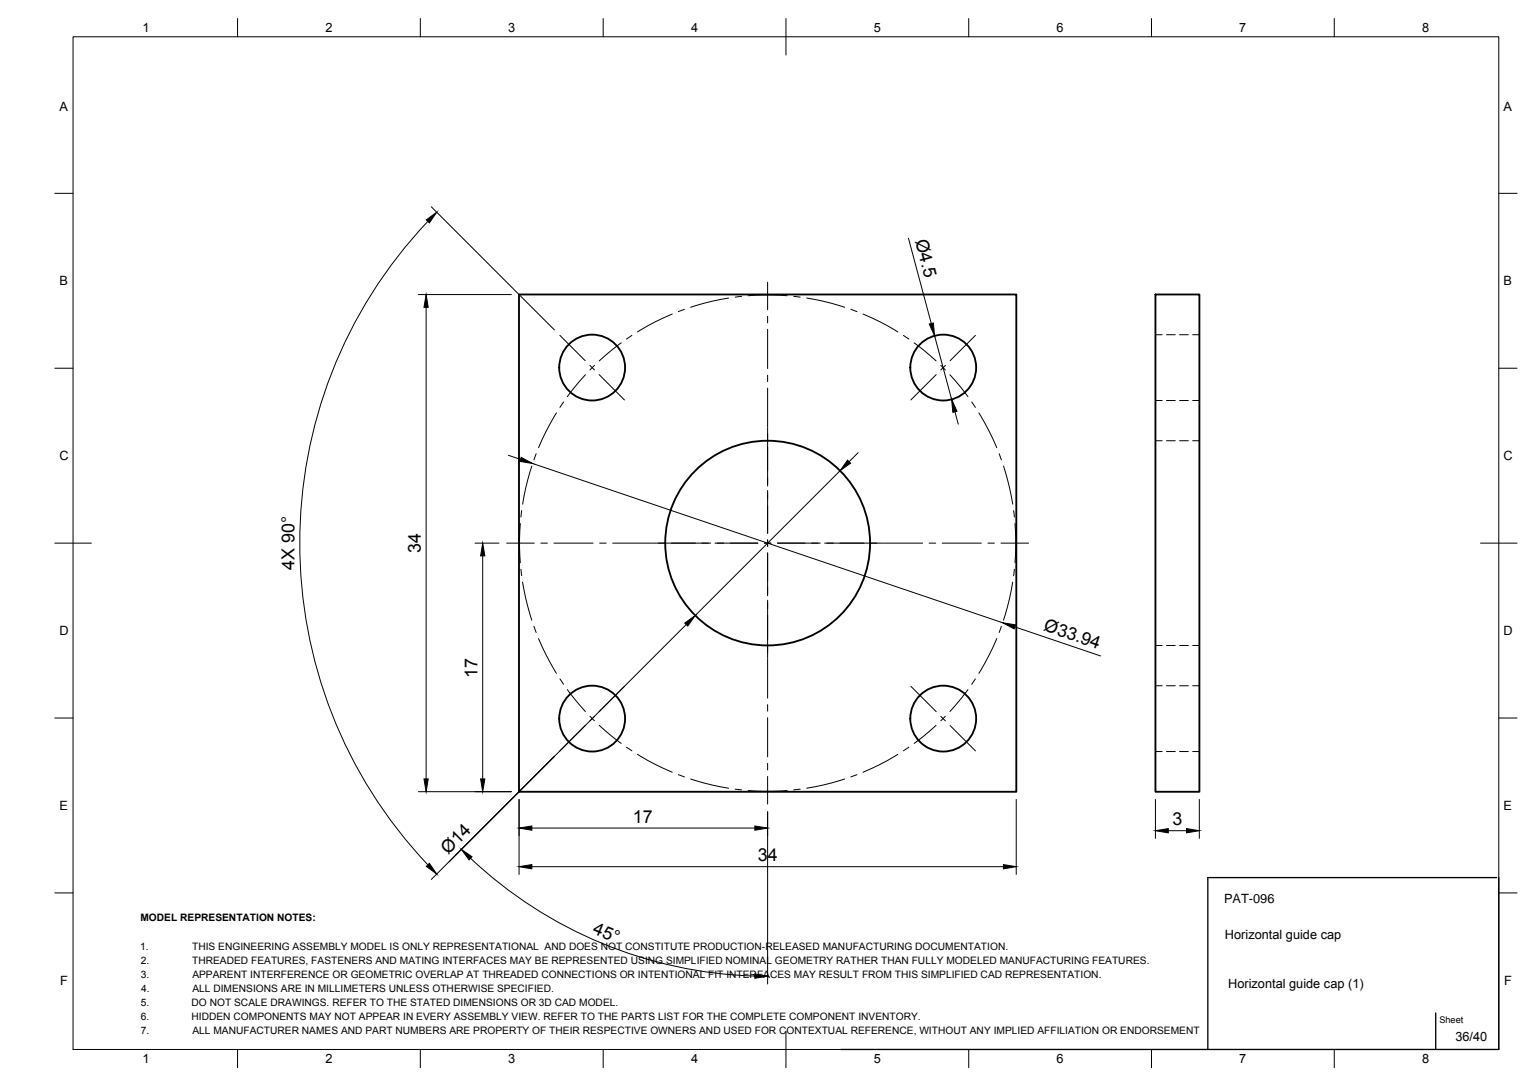
ISO-10303-21;
HEADER;
/* Generated by software containing ST-Developer
 * from STEP Tools, Inc. (www.steptools.com) 
 */

FILE_DESCRIPTION(
/* description */ ('PAT-096'),
/* implementation_level */ '2;1');

FILE_NAME(
/* name */ 'Horizontal guide cap.step',
/* time_stamp */ '2026-10-29T17:03:14-07:00',
/* author */ (''),
/* organization */ (''),
/* preprocessor_version */ 'ST-DEVELOPER v20.2',
/* originating_system */ 'Autodesk Translation Framework v15.17.0.0',
/* authorisation */ '');

FILE_SCHEMA (('AUTOMOTIVE_DESIGN { 1 0 10303 214 3 1 1 }'));
ENDSEC;

DATA;
#10=MECHANICAL_DESIGN_GEOMETRIC_PRESENTATION_REPRESENTATION('',(#433),#10650);
#363=SHAPE_REPRESENTATION_RELATIONSHIP('SRR','None',#10828,#394);
#394=ADVANCED_BREP_SHAPE_REPRESENTATION('',(#470),#10646);
#433=STYLED_ITEM('',(#11057),#470);
#470=MANIFOLD_SOLID_BREP('Body1',#5568);
#597=FACE_BOUND('',#1558,.T.);
#598=FACE_BOUND('',#1559,.T.);
#599=FACE_BOUND('',#1560,.T.);
#600=FACE_BOUND('',#1561,.T.);
#601=FACE_BOUND('',#1562,.T.);
#602=FACE_BOUND('',#1565,.T.);
#603=FACE_BOUND('',#1566,.T.);
#604=FACE_BOUND('',#1567,.T.);
#605=FACE_BOUND('',#1568,.T.);
#606=FACE_BOUND('',#1569,.T.);
#769=PLANE('',#6570);
#770=PLANE('',#6571);
#771=PLANE('',#6572);
#772=PLANE('',#6573);
#773=PLANE('',#6574);
#774=PLANE('',#6575);
#1091=FACE_OUTER_BOUND('',#1551,.T.);
#1092=FACE_OUTER_BOUND('',#1552,.T.);
#1093=FACE_OUTER_BOUND('',#1553,.T.);
#1094=FACE_OUTER_BOUND('',#1554,.T.);
#1095=FACE_OUTER_BOUND('',#1555,.T.);
#1096=FACE_OUTER_BOUND('',#1556,.T.);
#1097=FACE_OUTER_BOUND('',#1557,.T.);
#1098=FACE_OUTER_BOUND('',#1563,.T.);
#1099=FACE_OUTER_BOUND('',#1564,.T.);
#1100=FACE_OUTER_BOUND('',#1570,.T.);
#1101=FACE_OUTER_BOUND('',#1571,.T.);
#1551=EDGE_LOOP('',(#4935,#4936,#4937,#4938));
#1552=EDGE_LOOP('',(#4939,#4940,#4941,#4942));
#1553=EDGE_LOOP('',(#4943,#4944,#4945,#4946));
#1554=EDGE_LOOP('',(#4947,#4948,#4949,#4950));
#1555=EDGE_LOOP('',(#4951,#4952,#4953,#4954));
#1556=EDGE_LOOP('',(#4955,#4956,#4957,#4958));
#1557=EDGE_LOOP('',(#4959,#4960,#4961,#4962));
#1558=EDGE_LOOP('',(#4963));
#1559=EDGE_LOOP('',(#4964));
#1560=EDGE_LOOP('',(#4965));
#1561=EDGE_LOOP('',(#4966));
#1562=EDGE_LOOP('',(#4967));
#1563=EDGE_LOOP('',(#4968,#4969,#4970,#4971));
#1564=EDGE_LOOP('',(#4972,#4973,#4974,#4975));
#1565=EDGE_LOOP('',(#4976));
#1566=EDGE_LOOP('',(#4977));
#1567=EDGE_LOOP('',(#4978));
#1568=EDGE_LOOP('',(#4979));
#1569=EDGE_LOOP('',(#4980));
#1570=EDGE_LOOP('',(#4981,#4982,#4983,#4984));
#1571=EDGE_LOOP('',(#4985,#4986,#4987,#4988));
#1886=LINE('',#10372,#2215);
#1887=LINE('',#10378,#2216);
#1888=LINE('',#10384,#2217);
#1889=LINE('',#10390,#2218);
#1890=LINE('',#10396,#2219);
#1891=LINE('',#10401,#2220);
#1892=LINE('',#10403,#2221);
#1893=LINE('',#10405,#2222);
#1894=LINE('',#10406,#2223);
#1895=LINE('',#10409,#2224);
#1896=LINE('',#10411,#2225);
#1897=LINE('',#10412,#2226);
#1898=LINE('',#10415,#2227);
#1899=LINE('',#10417,#2228);
#1900=LINE('',#10418,#2229);
#1901=LINE('',#10420,#2230);
#1902=LINE('',#10421,#2231);
#2215=VECTOR('',#8240,0.225);
#2216=VECTOR('',#8247,0.225);
#2217=VECTOR('',#8254,0.225);
#2218=VECTOR('',#8261,0.225);
#2219=VECTOR('',#8268,0.7);
#2220=VECTOR('',#8273,1.);
#2221=VECTOR('',#8274,1.);
#2222=VECTOR('',#8275,1.);
#2223=VECTOR('',#8276,1.);
#2224=VECTOR('',#8279,1.);
#2225=VECTOR('',#8280,1.);
#2226=VECTOR('',#8281,1.);
#2227=VECTOR('',#8284,1.);
#2228=VECTOR('',#8285,1.);
#2229=VECTOR('',#8286,1.);
#2230=VECTOR('',#8289,1.);
#2231=VECTOR('',#8290,1.);
#2553=CIRCLE('',#6556,0.225);
#2554=CIRCLE('',#6557,0.225);
#2555=CIRCLE('',#6559,0.225);
#2556=CIRCLE('',#6560,0.225);
#2557=CIRCLE('',#6562,0.225);
#2558=CIRCLE('',#6563,0.225);
#2559=CIRCLE('',#6565,0.225);
#2560=CIRCLE('',#6566,0.225);
#2561=CIRCLE('',#6568,0.7);
#2562=CIRCLE('',#6569,0.7);
#2991=VERTEX_POINT('',#10369);
#2992=VERTEX_POINT('',#10371);
#2993=VERTEX_POINT('',#10375);
#2994=VERTEX_POINT('',#10377);
#2995=VERTEX_POINT('',#10381);
#2996=VERTEX_POINT('',#10383);
#2997=VERTEX_POINT('',#10387);
#2998=VERTEX_POINT('',#10389);
#2999=VERTEX_POINT('',#10393);
#3000=VERTEX_POINT('',#10395);
#3001=VERTEX_POINT('',#10399);
#3002=VERTEX_POINT('',#10400);
#3003=VERTEX_POINT('',#10402);
#3004=VERTEX_POINT('',#10404);
#3005=VERTEX_POINT('',#10408);
#3006=VERTEX_POINT('',#10410);
#3007=VERTEX_POINT('',#10414);
#3008=VERTEX_POINT('',#10416);
#3646=EDGE_CURVE('',#2991,#2991,#2553,.T.);
#3647=EDGE_CURVE('',#2991,#2992,#1886,.T.);
#3648=EDGE_CURVE('',#2992,#2992,#2554,.T.);
#3649=EDGE_CURVE('',#2993,#2993,#2555,.T.);
#3650=EDGE_CURVE('',#2993,#2994,#1887,.T.);
#3651=EDGE_CURVE('',#2994,#2994,#2556,.T.);
#3652=EDGE_CURVE('',#2995,#2995,#2557,.T.);
#3653=EDGE_CURVE('',#2995,#2996,#1888,.T.);
#3654=EDGE_CURVE('',#2996,#2996,#2558,.T.);
#3655=EDGE_CURVE('',#2997,#2997,#2559,.T.);
#3656=EDGE_CURVE('',#2997,#2998,#1889,.T.);
#3657=EDGE_CURVE('',#2998,#2998,#2560,.T.);
#3658=EDGE_CURVE('',#2999,#2999,#2561,.T.);
#3659=EDGE_CURVE('',#2999,#3000,#1890,.T.);
#3660=EDGE_CURVE('',#3000,#3000,#2562,.T.);
#3661=EDGE_CURVE('',#3001,#3002,#1891,.T.);
#3662=EDGE_CURVE('',#3002,#3003,#1892,.T.);
#3663=EDGE_CURVE('',#3004,#3003,#1893,.T.);
#3664=EDGE_CURVE('',#3001,#3004,#1894,.T.);
#3665=EDGE_CURVE('',#3005,#3001,#1895,.T.);
#3666=EDGE_CURVE('',#3006,#3004,#1896,.T.);
#3667=EDGE_CURVE('',#3005,#3006,#1897,.T.);
#3668=EDGE_CURVE('',#3007,#3005,#1898,.T.);
#3669=EDGE_CURVE('',#3008,#3006,#1899,.T.);
#3670=EDGE_CURVE('',#3007,#3008,#1900,.T.);
#3671=EDGE_CURVE('',#3002,#3007,#1901,.T.);
#3672=EDGE_CURVE('',#3003,#3008,#1902,.T.);
#4935=ORIENTED_EDGE('',*,*,#3646,.F.);
#4936=ORIENTED_EDGE('',*,*,#3647,.T.);
#4937=ORIENTED_EDGE('',*,*,#3648,.F.);
#4938=ORIENTED_EDGE('',*,*,#3647,.F.);
#4939=ORIENTED_EDGE('',*,*,#3649,.F.);
#4940=ORIENTED_EDGE('',*,*,#3650,.T.);
#4941=ORIENTED_EDGE('',*,*,#3651,.F.);
#4942=ORIENTED_EDGE('',*,*,#3650,.F.);
#4943=ORIENTED_EDGE('',*,*,#3652,.F.);
#4944=ORIENTED_EDGE('',*,*,#3653,.T.);
#4945=ORIENTED_EDGE('',*,*,#3654,.F.);
#4946=ORIENTED_EDGE('',*,*,#3653,.F.);
#4947=ORIENTED_EDGE('',*,*,#3655,.F.);
#4948=ORIENTED_EDGE('',*,*,#3656,.T.);
#4949=ORIENTED_EDGE('',*,*,#3657,.F.);
#4950=ORIENTED_EDGE('',*,*,#3656,.F.);
#4951=ORIENTED_EDGE('',*,*,#3658,.F.);
#4952=ORIENTED_EDGE('',*,*,#3659,.T.);
#4953=ORIENTED_EDGE('',*,*,#3660,.F.);
#4954=ORIENTED_EDGE('',*,*,#3659,.F.);
#4955=ORIENTED_EDGE('',*,*,#3661,.T.);
#4956=ORIENTED_EDGE('',*,*,#3662,.T.);
#4957=ORIENTED_EDGE('',*,*,#3663,.F.);
#4958=ORIENTED_EDGE('',*,*,#3664,.F.);
#4959=ORIENTED_EDGE('',*,*,#3665,.T.);
#4960=ORIENTED_EDGE('',*,*,#3664,.T.);
#4961=ORIENTED_EDGE('',*,*,#3666,.F.);
#4962=ORIENTED_EDGE('',*,*,#3667,.F.);
#4963=ORIENTED_EDGE('',*,*,#3660,.T.);
#4964=ORIENTED_EDGE('',*,*,#3657,.T.);
#4965=ORIENTED_EDGE('',*,*,#3654,.T.);
#4966=ORIENTED_EDGE('',*,*,#3651,.T.);
#4967=ORIENTED_EDGE('',*,*,#3648,.T.);
#4968=ORIENTED_EDGE('',*,*,#3668,.T.);
#4969=ORIENTED_EDGE('',*,*,#3667,.T.);
#4970=ORIENTED_EDGE('',*,*,#3669,.F.);
#4971=ORIENTED_EDGE('',*,*,#3670,.F.);
#4972=ORIENTED_EDGE('',*,*,#3671,.T.);
#4973=ORIENTED_EDGE('',*,*,#3670,.T.);
#4974=ORIENTED_EDGE('',*,*,#3672,.F.);
#4975=ORIENTED_EDGE('',*,*,#3662,.F.);
#4976=ORIENTED_EDGE('',*,*,#3658,.T.);
#4977=ORIENTED_EDGE('',*,*,#3655,.T.);
#4978=ORIENTED_EDGE('',*,*,#3652,.T.);
#4979=ORIENTED_EDGE('',*,*,#3649,.T.);
#4980=ORIENTED_EDGE('',*,*,#3646,.T.);
#4981=ORIENTED_EDGE('',*,*,#3672,.T.);
#4982=ORIENTED_EDGE('',*,*,#3669,.T.);
#4983=ORIENTED_EDGE('',*,*,#3666,.T.);
#4984=ORIENTED_EDGE('',*,*,#3663,.T.);
#4985=ORIENTED_EDGE('',*,*,#3671,.F.);
#4986=ORIENTED_EDGE('',*,*,#3661,.F.);
#4987=ORIENTED_EDGE('',*,*,#3665,.F.);
#4988=ORIENTED_EDGE('',*,*,#3668,.F.);
#5184=CYLINDRICAL_SURFACE('',#6555,0.225);
#5185=CYLINDRICAL_SURFACE('',#6558,0.225);
#5186=CYLINDRICAL_SURFACE('',#6561,0.225);
#5187=CYLINDRICAL_SURFACE('',#6564,0.225);
#5188=CYLINDRICAL_SURFACE('',#6567,0.7);
#5496=ADVANCED_FACE('',(#1091),#5184,.F.);
#5497=ADVANCED_FACE('',(#1092),#5185,.F.);
#5498=ADVANCED_FACE('',(#1093),#5186,.F.);
#5499=ADVANCED_FACE('',(#1094),#5187,.F.);
#5500=ADVANCED_FACE('',(#1095),#5188,.F.);
#5501=ADVANCED_FACE('',(#1096),#769,.T.);
#5502=ADVANCED_FACE('',(#1097,#597,#598,#599,#600,#601),#770,.T.);
#5503=ADVANCED_FACE('',(#1098),#771,.T.);
#5504=ADVANCED_FACE('',(#1099,#602,#603,#604,#605,#606),#772,.T.);
#5505=ADVANCED_FACE('',(#1100),#773,.T.);
#5506=ADVANCED_FACE('',(#1101),#774,.F.);
#5568=CLOSED_SHELL('',(#5496,#5497,#5498,#5499,#5500,#5501,#5502,#5503,
#5504,#5505,#5506));
#6554=AXIS2_PLACEMENT_3D('',#10367,#8234,#8235);
#6555=AXIS2_PLACEMENT_3D('',#10368,#8236,#8237);
#6556=AXIS2_PLACEMENT_3D('',#10370,#8238,#8239);
#6557=AXIS2_PLACEMENT_3D('',#10373,#8241,#8242);
#6558=AXIS2_PLACEMENT_3D('',#10374,#8243,#8244);
#6559=AXIS2_PLACEMENT_3D('',#10376,#8245,#8246);
#6560=AXIS2_PLACEMENT_3D('',#10379,#8248,#8249);
#6561=AXIS2_PLACEMENT_3D('',#10380,#8250,#8251);
#6562=AXIS2_PLACEMENT_3D('',#10382,#8252,#8253);
#6563=AXIS2_PLACEMENT_3D('',#10385,#8255,#8256);
#6564=AXIS2_PLACEMENT_3D('',#10386,#8257,#8258);
#6565=AXIS2_PLACEMENT_3D('',#10388,#8259,#8260);
#6566=AXIS2_PLACEMENT_3D('',#10391,#8262,#8263);
#6567=AXIS2_PLACEMENT_3D('',#10392,#8264,#8265);
#6568=AXIS2_PLACEMENT_3D('',#10394,#8266,#8267);
#6569=AXIS2_PLACEMENT_3D('',#10397,#8269,#8270);
#6570=AXIS2_PLACEMENT_3D('',#10398,#8271,#8272);
#6571=AXIS2_PLACEMENT_3D('',#10407,#8277,#8278);
#6572=AXIS2_PLACEMENT_3D('',#10413,#8282,#8283);
#6573=AXIS2_PLACEMENT_3D('',#10419,#8287,#8288);
#6574=AXIS2_PLACEMENT_3D('',#10422,#8291,#8292);
#6575=AXIS2_PLACEMENT_3D('',#10423,#8293,#8294);
#8234=DIRECTION('axis',(0.,0.,1.));
#8235=DIRECTION('refdir',(1.,0.,0.));
#8236=DIRECTION('center_axis',(1.,0.,0.));
#8237=DIRECTION('ref_axis',(0.,0.,-1.));
#8238=DIRECTION('center_axis',(1.,0.,0.));
#8239=DIRECTION('ref_axis',(0.,0.,-1.));
#8240=DIRECTION('',(1.,0.,0.));
#8241=DIRECTION('center_axis',(-1.,0.,0.));
#8242=DIRECTION('ref_axis',(0.,0.,-1.));
#8243=DIRECTION('center_axis',(1.,0.,0.));
#8244=DIRECTION('ref_axis',(0.,0.,-1.));
#8245=DIRECTION('center_axis',(1.,0.,0.));
#8246=DIRECTION('ref_axis',(0.,0.,-1.));
#8247=DIRECTION('',(1.,0.,0.));
#8248=DIRECTION('center_axis',(-1.,0.,0.));
#8249=DIRECTION('ref_axis',(0.,0.,-1.));
#8250=DIRECTION('center_axis',(1.,0.,0.));
#8251=DIRECTION('ref_axis',(0.,0.,-1.));
#8252=DIRECTION('center_axis',(1.,0.,0.));
#8253=DIRECTION('ref_axis',(0.,0.,-1.));
#8254=DIRECTION('',(1.,0.,0.));
#8255=DIRECTION('center_axis',(-1.,0.,0.));
#8256=DIRECTION('ref_axis',(0.,0.,-1.));
#8257=DIRECTION('center_axis',(1.,0.,0.));
#8258=DIRECTION('ref_axis',(0.,0.,-1.));
#8259=DIRECTION('center_axis',(1.,0.,0.));
#8260=DIRECTION('ref_axis',(0.,0.,-1.));
#8261=DIRECTION('',(1.,0.,0.));
#8262=DIRECTION('center_axis',(-1.,0.,0.));
#8263=DIRECTION('ref_axis',(0.,0.,-1.));
#8264=DIRECTION('center_axis',(1.,0.,0.));
#8265=DIRECTION('ref_axis',(0.,0.,-1.));
#8266=DIRECTION('center_axis',(1.,0.,0.));
#8267=DIRECTION('ref_axis',(0.,0.,-1.));
#8268=DIRECTION('',(1.,0.,0.));
#8269=DIRECTION('center_axis',(-1.,0.,0.));
#8270=DIRECTION('ref_axis',(0.,0.,-1.));
#8271=DIRECTION('center_axis',(0.,1.,0.));
#8272=DIRECTION('ref_axis',(-1.,0.,0.));
#8273=DIRECTION('',(-1.,0.,0.));
#8274=DIRECTION('',(0.,0.,1.));
#8275=DIRECTION('',(-1.,0.,0.));
#8276=DIRECTION('',(0.,0.,1.));
#8277=DIRECTION('center_axis',(1.,0.,0.));
#8278=DIRECTION('ref_axis',(0.,1.,0.));
#8279=DIRECTION('',(0.,1.,0.));
#8280=DIRECTION('',(0.,1.,0.));
#8281=DIRECTION('',(0.,0.,1.));
#8282=DIRECTION('center_axis',(0.,-1.,0.));
#8283=DIRECTION('ref_axis',(1.,0.,0.));
#8284=DIRECTION('',(1.,0.,0.));
#8285=DIRECTION('',(1.,0.,0.));
#8286=DIRECTION('',(0.,0.,1.));
#8287=DIRECTION('center_axis',(-1.,0.,0.));
#8288=DIRECTION('ref_axis',(0.,-1.,0.));
#8289=DIRECTION('',(0.,-1.,0.));
#8290=DIRECTION('',(0.,-1.,0.));
#8291=DIRECTION('center_axis',(0.,0.,1.));
#8292=DIRECTION('ref_axis',(1.,0.,0.));
#8293=DIRECTION('center_axis',(0.,0.,1.));
#8294=DIRECTION('ref_axis',(1.,0.,0.));
#10367=CARTESIAN_POINT('',(0.,0.,0.));
#10368=CARTESIAN_POINT('Origin',(8.1,3.2,2.8));
#10369=CARTESIAN_POINT('',(8.2,3.2,3.025));
#10370=CARTESIAN_POINT('Origin',(8.2,3.2,2.8));
#10371=CARTESIAN_POINT('',(8.5,3.2,3.025));
#10372=CARTESIAN_POINT('',(8.1,3.2,3.025));
#10373=CARTESIAN_POINT('Origin',(8.5,3.2,2.8));
#10374=CARTESIAN_POINT('Origin',(8.1,0.8,5.2));
#10375=CARTESIAN_POINT('',(8.2,0.8,5.425));
#10376=CARTESIAN_POINT('Origin',(8.2,0.8,5.2));
#10377=CARTESIAN_POINT('',(8.5,0.8,5.425));
#10378=CARTESIAN_POINT('',(8.1,0.8,5.425));
#10379=CARTESIAN_POINT('Origin',(8.5,0.8,5.2));
#10380=CARTESIAN_POINT('Origin',(8.1,0.8,2.8));
#10381=CARTESIAN_POINT('',(8.2,0.8,3.025));
#10382=CARTESIAN_POINT('Origin',(8.2,0.8,2.8));
#10383=CARTESIAN_POINT('',(8.5,0.8,3.025));
#10384=CARTESIAN_POINT('',(8.1,0.8,3.025));
#10385=CARTESIAN_POINT('Origin',(8.5,0.8,2.8));
#10386=CARTESIAN_POINT('Origin',(8.1,3.2,5.2));
#10387=CARTESIAN_POINT('',(8.2,3.2,5.425));
#10388=CARTESIAN_POINT('Origin',(8.2,3.2,5.2));
#10389=CARTESIAN_POINT('',(8.5,3.2,5.425));
#10390=CARTESIAN_POINT('',(8.1,3.2,5.425));
#10391=CARTESIAN_POINT('Origin',(8.5,3.2,5.2));
#10392=CARTESIAN_POINT('Origin',(8.1,2.,4.));
#10393=CARTESIAN_POINT('',(8.2,2.,4.7));
#10394=CARTESIAN_POINT('Origin',(8.2,2.,4.));
#10395=CARTESIAN_POINT('',(8.5,2.,4.7));
#10396=CARTESIAN_POINT('',(8.1,2.,4.7));
#10397=CARTESIAN_POINT('Origin',(8.5,2.,4.));
#10398=CARTESIAN_POINT('Origin',(8.5,3.7,2.3));
#10399=CARTESIAN_POINT('',(8.5,3.7,2.3));
#10400=CARTESIAN_POINT('',(8.2,3.7,2.3));
#10401=CARTESIAN_POINT('',(8.5,3.7,2.3));
#10402=CARTESIAN_POINT('',(8.2,3.7,5.7));
#10403=CARTESIAN_POINT('',(8.2,3.7,2.3));
#10404=CARTESIAN_POINT('',(8.5,3.7,5.7));
#10405=CARTESIAN_POINT('',(8.5,3.7,5.7));
#10406=CARTESIAN_POINT('',(8.5,3.7,2.3));
#10407=CARTESIAN_POINT('Origin',(8.5,0.3,2.3));
#10408=CARTESIAN_POINT('',(8.5,0.3,2.3));
#10409=CARTESIAN_POINT('',(8.5,0.3,2.3));
#10410=CARTESIAN_POINT('',(8.5,0.3,5.7));
#10411=CARTESIAN_POINT('',(8.5,0.3,5.7));
#10412=CARTESIAN_POINT('',(8.5,0.3,2.3));
#10413=CARTESIAN_POINT('Origin',(8.2,0.3,2.3));
#10414=CARTESIAN_POINT('',(8.2,0.3,2.3));
#10415=CARTESIAN_POINT('',(8.2,0.3,2.3));
#10416=CARTESIAN_POINT('',(8.2,0.3,5.7));
#10417=CARTESIAN_POINT('',(8.2,0.3,5.7));
#10418=CARTESIAN_POINT('',(8.2,0.3,2.3));
#10419=CARTESIAN_POINT('Origin',(8.2,3.7,2.3));
#10420=CARTESIAN_POINT('',(8.2,3.7,2.3));
#10421=CARTESIAN_POINT('',(8.2,3.7,5.7));
#10422=CARTESIAN_POINT('Origin',(8.35,2.,5.7));
#10423=CARTESIAN_POINT('Origin',(8.35,2.,2.3));
#10607=UNCERTAINTY_MEASURE_WITH_UNIT(LENGTH_MEASURE(0.001),#10651,
'DISTANCE_ACCURACY_VALUE',
'Maximum model space distance between geometric entities at asserted c
onnectivities');
#10611=UNCERTAINTY_MEASURE_WITH_UNIT(LENGTH_MEASURE(0.001),#10651,
'DISTANCE_ACCURACY_VALUE',
'Maximum model space distance between geometric entities at asserted c
onnectivities');
#10646=(
GEOMETRIC_REPRESENTATION_CONTEXT(3)
GLOBAL_UNCERTAINTY_ASSIGNED_CONTEXT((#10607))
GLOBAL_UNIT_ASSIGNED_CONTEXT((#10651,#10653,#10654))
REPRESENTATION_CONTEXT('','3D')
);
#10650=(
GEOMETRIC_REPRESENTATION_CONTEXT(3)
GLOBAL_UNCERTAINTY_ASSIGNED_CONTEXT((#10611))
GLOBAL_UNIT_ASSIGNED_CONTEXT((#10651,#10653,#10654))
REPRESENTATION_CONTEXT('','3D')
);
#10651=(
LENGTH_UNIT()
NAMED_UNIT(*)
SI_UNIT(.CENTI.,.METRE.)
);
#10653=(
NAMED_UNIT(*)
PLANE_ANGLE_UNIT()
SI_UNIT($,.RADIAN.)
);
#10654=(
NAMED_UNIT(*)
SI_UNIT($,.STERADIAN.)
SOLID_ANGLE_UNIT()
);
#10689=SHAPE_DEFINITION_REPRESENTATION(#10737,#10828);
#10737=PRODUCT_DEFINITION_SHAPE('',$,#10867);
#10828=SHAPE_REPRESENTATION('',(#6554),#10646);
#10832=PRODUCT_DEFINITION_CONTEXT('part definition',#10948,'design');
#10867=PRODUCT_DEFINITION('Horizontal guide cap','Horizontal guide cap',
#10905,#10832);
#10905=PRODUCT_DEFINITION_FORMATION('',$,#10984);
#10948=APPLICATION_CONTEXT(
'Core Data for Automotive Mechanical Design Process');
#10949=PRODUCT_CONTEXT('part definition',#10948,'mechanical');
#10984=PRODUCT('Horizontal guide cap','Horizontal guide cap',
'Horizontal guide cap',(#10949));
#11051=COLOUR_RGB('Sky Blue',0.24,0.69,0.87);
#11052=FILL_AREA_STYLE_COLOUR('',#11051);
#11053=FILL_AREA_STYLE('',(#11052));
#11054=SURFACE_STYLE_FILL_AREA(#11053);
#11055=SURFACE_SIDE_STYLE('',(#11054));
#11056=SURFACE_STYLE_USAGE(.BOTH.,#11055);
#11057=PRESENTATION_STYLE_ASSIGNMENT((#11056));
ENDSEC;
END-ISO-10303-21;
